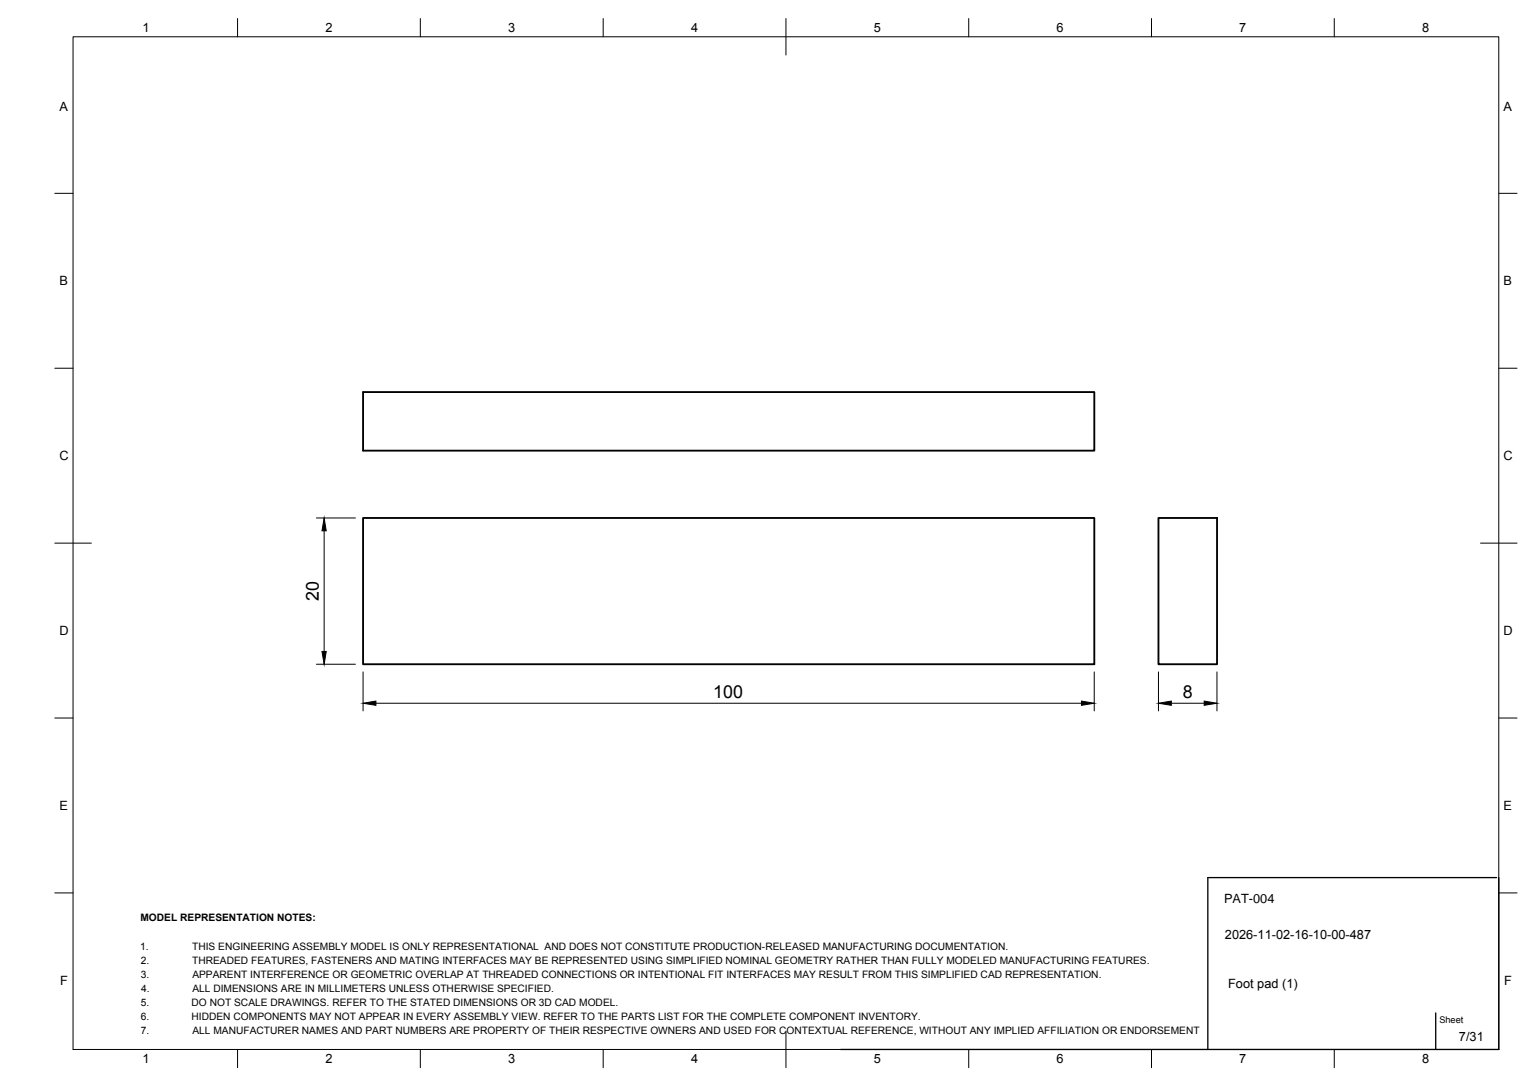
ISO-10303-21;
HEADER;
/* Generated by software containing ST-Developer
 * from STEP Tools, Inc. (www.steptools.com) 
 */

FILE_DESCRIPTION(
/* description */ ('Air blow-off nozzle station'),
/* implementation_level */ '2;1');

FILE_NAME(
/* name */ 'Foot pad (1).step',
/* time_stamp */ '2026-10-27T10:53:54-07:00',
/* author */ (''),
/* organization */ (''),
/* preprocessor_version */ 'ST-DEVELOPER v20.2',
/* originating_system */ 'Autodesk Translation Framework v15.17.0.0',
/* authorisation */ '');

FILE_SCHEMA (('AUTOMOTIVE_DESIGN { 1 0 10303 214 3 1 1 }'));
ENDSEC;

DATA;
#10=MECHANICAL_DESIGN_GEOMETRIC_PRESENTATION_REPRESENTATION('',(#239),#7897);
#189=SHAPE_REPRESENTATION_RELATIONSHIP('SRR','None',#8003,#214);
#214=ADVANCED_BREP_SHAPE_REPRESENTATION('',(#264),#7870);
#239=STYLED_ITEM('',(#8213),#264);
#264=MANIFOLD_SOLID_BREP('Body1',#4288);
#383=PLANE('',#4609);
#384=PLANE('',#4610);
#385=PLANE('',#4611);
#386=PLANE('',#4612);
#387=PLANE('',#4613);
#388=PLANE('',#4614);
#553=FACE_OUTER_BOUND('',#811,.T.);
#554=FACE_OUTER_BOUND('',#812,.T.);
#555=FACE_OUTER_BOUND('',#813,.T.);
#556=FACE_OUTER_BOUND('',#814,.T.);
#557=FACE_OUTER_BOUND('',#815,.T.);
#558=FACE_OUTER_BOUND('',#816,.T.);
#811=EDGE_LOOP('',(#2951,#2952,#2953,#2954));
#812=EDGE_LOOP('',(#2955,#2956,#2957,#2958));
#813=EDGE_LOOP('',(#2959,#2960,#2961,#2962));
#814=EDGE_LOOP('',(#2963,#2964,#2965,#2966));
#815=EDGE_LOOP('',(#2967,#2968,#2969,#2970));
#816=EDGE_LOOP('',(#2971,#2972,#2973,#2974));
#1163=LINE('',#6458,#1517);
#1164=LINE('',#6460,#1518);
#1165=LINE('',#6462,#1519);
#1166=LINE('',#6463,#1520);
#1167=LINE('',#6466,#1521);
#1168=LINE('',#6468,#1522);
#1169=LINE('',#6469,#1523);
#1170=LINE('',#6472,#1524);
#1171=LINE('',#6474,#1525);
#1172=LINE('',#6475,#1526);
#1173=LINE('',#6477,#1527);
#1174=LINE('',#6478,#1528);
#1517=VECTOR('',#5139,1.);
#1518=VECTOR('',#5140,1.);
#1519=VECTOR('',#5141,1.);
#1520=VECTOR('',#5142,1.);
#1521=VECTOR('',#5145,1.);
#1522=VECTOR('',#5146,1.);
#1523=VECTOR('',#5147,1.);
#1524=VECTOR('',#5150,1.);
#1525=VECTOR('',#5151,1.);
#1526=VECTOR('',#5152,1.);
#1527=VECTOR('',#5155,1.);
#1528=VECTOR('',#5156,1.);
#2025=VERTEX_POINT('',#6456);
#2026=VERTEX_POINT('',#6457);
#2027=VERTEX_POINT('',#6459);
#2028=VERTEX_POINT('',#6461);
#2029=VERTEX_POINT('',#6465);
#2030=VERTEX_POINT('',#6467);
#2031=VERTEX_POINT('',#6471);
#2032=VERTEX_POINT('',#6473);
#2393=EDGE_CURVE('',#2025,#2026,#1163,.T.);
#2394=EDGE_CURVE('',#2026,#2027,#1164,.T.);
#2395=EDGE_CURVE('',#2028,#2027,#1165,.T.);
#2396=EDGE_CURVE('',#2025,#2028,#1166,.T.);
#2397=EDGE_CURVE('',#2029,#2025,#1167,.T.);
#2398=EDGE_CURVE('',#2030,#2028,#1168,.T.);
#2399=EDGE_CURVE('',#2029,#2030,#1169,.T.);
#2400=EDGE_CURVE('',#2031,#2029,#1170,.T.);
#2401=EDGE_CURVE('',#2032,#2030,#1171,.T.);
#2402=EDGE_CURVE('',#2031,#2032,#1172,.T.);
#2403=EDGE_CURVE('',#2026,#2031,#1173,.T.);
#2404=EDGE_CURVE('',#2027,#2032,#1174,.T.);
#2951=ORIENTED_EDGE('',*,*,#2393,.T.);
#2952=ORIENTED_EDGE('',*,*,#2394,.T.);
#2953=ORIENTED_EDGE('',*,*,#2395,.F.);
#2954=ORIENTED_EDGE('',*,*,#2396,.F.);
#2955=ORIENTED_EDGE('',*,*,#2397,.T.);
#2956=ORIENTED_EDGE('',*,*,#2396,.T.);
#2957=ORIENTED_EDGE('',*,*,#2398,.F.);
#2958=ORIENTED_EDGE('',*,*,#2399,.F.);
#2959=ORIENTED_EDGE('',*,*,#2400,.T.);
#2960=ORIENTED_EDGE('',*,*,#2399,.T.);
#2961=ORIENTED_EDGE('',*,*,#2401,.F.);
#2962=ORIENTED_EDGE('',*,*,#2402,.F.);
#2963=ORIENTED_EDGE('',*,*,#2403,.T.);
#2964=ORIENTED_EDGE('',*,*,#2402,.T.);
#2965=ORIENTED_EDGE('',*,*,#2404,.F.);
#2966=ORIENTED_EDGE('',*,*,#2394,.F.);
#2967=ORIENTED_EDGE('',*,*,#2404,.T.);
#2968=ORIENTED_EDGE('',*,*,#2401,.T.);
#2969=ORIENTED_EDGE('',*,*,#2398,.T.);
#2970=ORIENTED_EDGE('',*,*,#2395,.T.);
#2971=ORIENTED_EDGE('',*,*,#2403,.F.);
#2972=ORIENTED_EDGE('',*,*,#2393,.F.);
#2973=ORIENTED_EDGE('',*,*,#2397,.F.);
#2974=ORIENTED_EDGE('',*,*,#2400,.F.);
#4043=ADVANCED_FACE('',(#553),#383,.T.);
#4044=ADVANCED_FACE('',(#554),#384,.T.);
#4045=ADVANCED_FACE('',(#555),#385,.T.);
#4046=ADVANCED_FACE('',(#556),#386,.T.);
#4047=ADVANCED_FACE('',(#557),#387,.T.);
#4048=ADVANCED_FACE('',(#558),#388,.F.);
#4288=CLOSED_SHELL('',(#4043,#4044,#4045,#4046,#4047,#4048));
#4608=AXIS2_PLACEMENT_3D('',#6454,#5135,#5136);
#4609=AXIS2_PLACEMENT_3D('',#6455,#5137,#5138);
#4610=AXIS2_PLACEMENT_3D('',#6464,#5143,#5144);
#4611=AXIS2_PLACEMENT_3D('',#6470,#5148,#5149);
#4612=AXIS2_PLACEMENT_3D('',#6476,#5153,#5154);
#4613=AXIS2_PLACEMENT_3D('',#6479,#5157,#5158);
#4614=AXIS2_PLACEMENT_3D('',#6480,#5159,#5160);
#5135=DIRECTION('axis',(0.,0.,1.));
#5136=DIRECTION('refdir',(1.,0.,0.));
#5137=DIRECTION('center_axis',(0.,1.,0.));
#5138=DIRECTION('ref_axis',(-1.,0.,0.));
#5139=DIRECTION('',(-1.,0.,0.));
#5140=DIRECTION('',(0.,0.,1.));
#5141=DIRECTION('',(-1.,0.,0.));
#5142=DIRECTION('',(0.,0.,1.));
#5143=DIRECTION('center_axis',(1.,0.,0.));
#5144=DIRECTION('ref_axis',(0.,1.,0.));
#5145=DIRECTION('',(0.,1.,0.));
#5146=DIRECTION('',(0.,1.,0.));
#5147=DIRECTION('',(0.,0.,1.));
#5148=DIRECTION('center_axis',(0.,-1.,0.));
#5149=DIRECTION('ref_axis',(1.,0.,0.));
#5150=DIRECTION('',(1.,0.,0.));
#5151=DIRECTION('',(1.,0.,0.));
#5152=DIRECTION('',(0.,0.,1.));
#5153=DIRECTION('center_axis',(-1.,0.,0.));
#5154=DIRECTION('ref_axis',(0.,-1.,0.));
#5155=DIRECTION('',(0.,-1.,0.));
#5156=DIRECTION('',(0.,-1.,0.));
#5157=DIRECTION('center_axis',(0.,0.,1.));
#5158=DIRECTION('ref_axis',(1.,0.,0.));
#5159=DIRECTION('center_axis',(0.,0.,1.));
#5160=DIRECTION('ref_axis',(1.,0.,0.));
#6454=CARTESIAN_POINT('',(0.,0.,0.));
#6455=CARTESIAN_POINT('Origin',(6.,6.,-0.8));
#6456=CARTESIAN_POINT('',(6.,6.,-0.8));
#6457=CARTESIAN_POINT('',(4.,6.,-0.8));
#6458=CARTESIAN_POINT('',(6.,6.,-0.8));
#6459=CARTESIAN_POINT('',(4.,6.,0.));
#6460=CARTESIAN_POINT('',(4.,6.,-0.8));
#6461=CARTESIAN_POINT('',(6.,6.,0.));
#6462=CARTESIAN_POINT('',(6.,6.,0.));
#6463=CARTESIAN_POINT('',(6.,6.,-0.8));
#6464=CARTESIAN_POINT('Origin',(6.,-4.,-0.8));
#6465=CARTESIAN_POINT('',(6.,-4.,-0.8));
#6466=CARTESIAN_POINT('',(6.,-4.,-0.8));
#6467=CARTESIAN_POINT('',(6.,-4.,0.));
#6468=CARTESIAN_POINT('',(6.,-4.,0.));
#6469=CARTESIAN_POINT('',(6.,-4.,-0.8));
#6470=CARTESIAN_POINT('Origin',(4.,-4.,-0.8));
#6471=CARTESIAN_POINT('',(4.,-4.,-0.8));
#6472=CARTESIAN_POINT('',(4.,-4.,-0.8));
#6473=CARTESIAN_POINT('',(4.,-4.,0.));
#6474=CARTESIAN_POINT('',(4.,-4.,0.));
#6475=CARTESIAN_POINT('',(4.,-4.,-0.8));
#6476=CARTESIAN_POINT('Origin',(4.,6.,-0.8));
#6477=CARTESIAN_POINT('',(4.,6.,-0.8));
#6478=CARTESIAN_POINT('',(4.,6.,0.));
#6479=CARTESIAN_POINT('Origin',(5.,1.,0.));
#6480=CARTESIAN_POINT('Origin',(5.,1.,-0.8));
#7838=UNCERTAINTY_MEASURE_WITH_UNIT(LENGTH_MEASURE(0.001),#7898,
'DISTANCE_ACCURACY_VALUE',
'Maximum model space distance between geometric entities at asserted c
onnectivities');
#7865=UNCERTAINTY_MEASURE_WITH_UNIT(LENGTH_MEASURE(0.001),#7898,
'DISTANCE_ACCURACY_VALUE',
'Maximum model space distance between geometric entities at asserted c
onnectivities');
#7870=(
GEOMETRIC_REPRESENTATION_CONTEXT(3)
GLOBAL_UNCERTAINTY_ASSIGNED_CONTEXT((#7838))
GLOBAL_UNIT_ASSIGNED_CONTEXT((#7898,#7900,#7901))
REPRESENTATION_CONTEXT('','3D')
);
#7897=(
GEOMETRIC_REPRESENTATION_CONTEXT(3)
GLOBAL_UNCERTAINTY_ASSIGNED_CONTEXT((#7865))
GLOBAL_UNIT_ASSIGNED_CONTEXT((#7898,#7900,#7901))
REPRESENTATION_CONTEXT('','3D')
);
#7898=(
LENGTH_UNIT()
NAMED_UNIT(*)
SI_UNIT(.CENTI.,.METRE.)
);
#7900=(
NAMED_UNIT(*)
PLANE_ANGLE_UNIT()
SI_UNIT($,.RADIAN.)
);
#7901=(
NAMED_UNIT(*)
SI_UNIT($,.STERADIAN.)
SOLID_ANGLE_UNIT()
);
#7906=SHAPE_DEFINITION_REPRESENTATION(#7937,#8003);
#7937=PRODUCT_DEFINITION_SHAPE('',$,#8035);
#8003=SHAPE_REPRESENTATION('',(#4608),#7870);
#8030=PRODUCT_DEFINITION_CONTEXT('part definition',#8125,'design');
#8035=PRODUCT_DEFINITION('Foot pad (1)','Foot pad (1)',#8066,#8030);
#8066=PRODUCT_DEFINITION_FORMATION('',$,#8131);
#8125=APPLICATION_CONTEXT(
'Core Data for Automotive Mechanical Design Process');
#8126=PRODUCT_CONTEXT('part definition',#8125,'mechanical');
#8131=PRODUCT('Foot pad (1)','Foot pad (1)','Foot pad (1)',(#8126));
#8207=COLOUR_RGB('Sky Blue',0.24,0.69,0.87);
#8208=FILL_AREA_STYLE_COLOUR('',#8207);
#8209=FILL_AREA_STYLE('',(#8208));
#8210=SURFACE_STYLE_FILL_AREA(#8209);
#8211=SURFACE_SIDE_STYLE('',(#8210));
#8212=SURFACE_STYLE_USAGE(.BOTH.,#8211);
#8213=PRESENTATION_STYLE_ASSIGNMENT((#8212));
ENDSEC;
END-ISO-10303-21;
